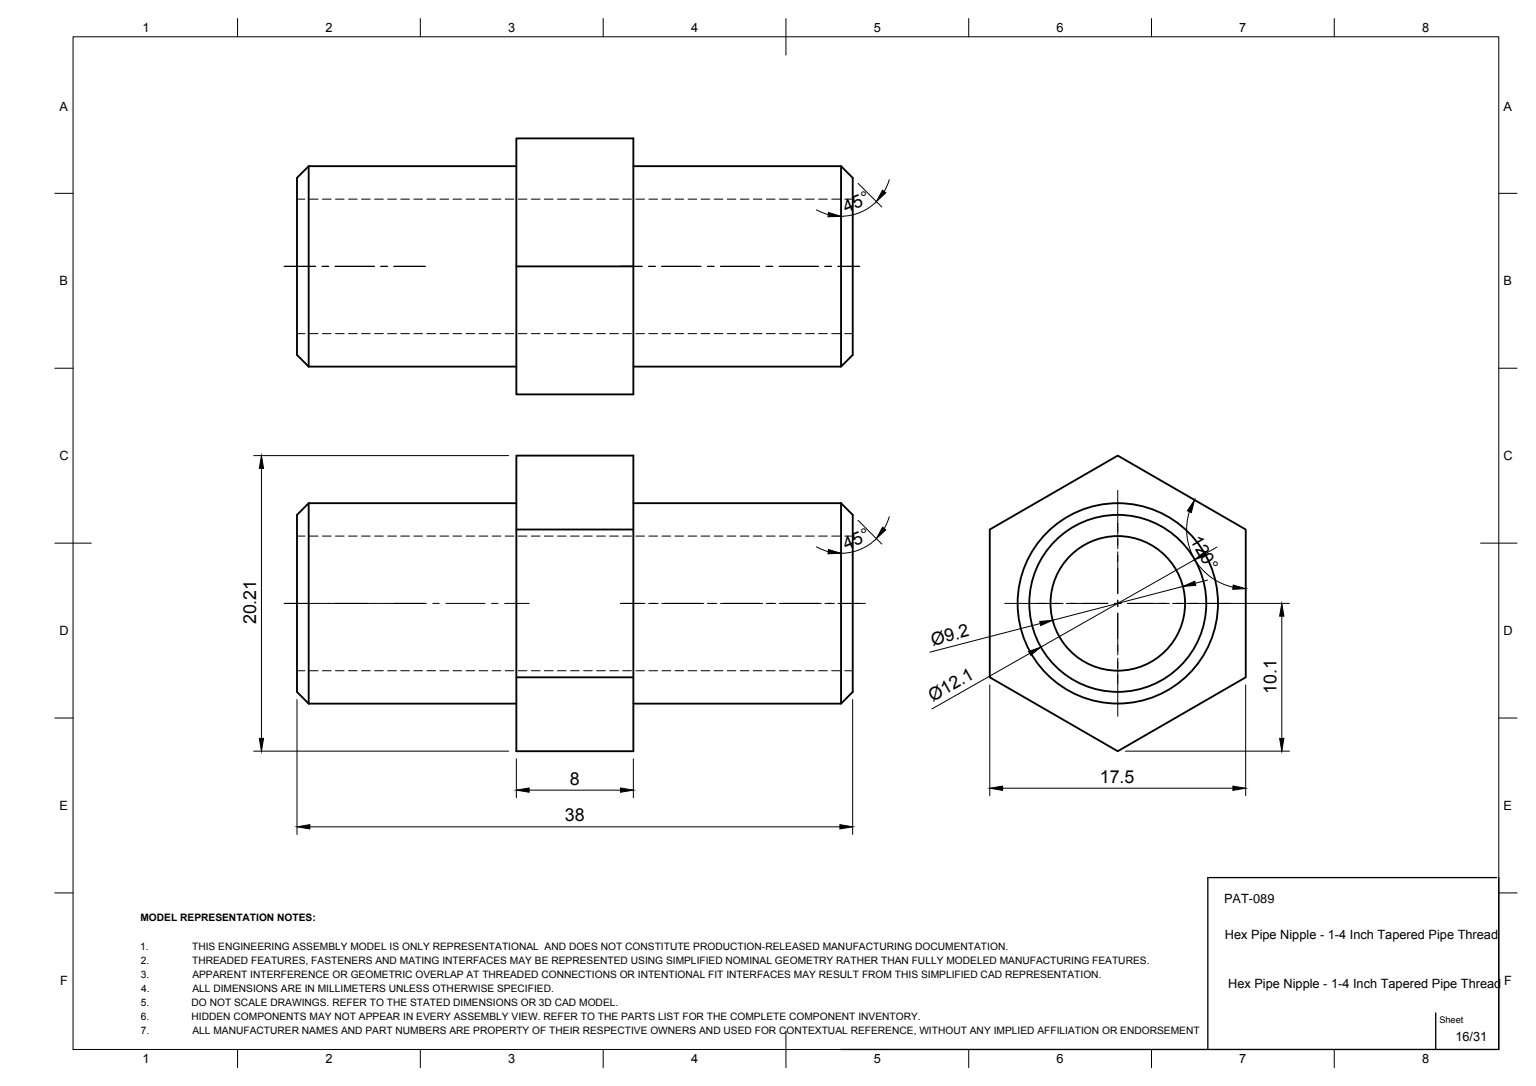
ISO-10303-21;
HEADER;
/* Generated by software containing ST-Developer
 * from STEP Tools, Inc. (www.steptools.com) 
 */

FILE_DESCRIPTION(
/* description */ ('Rotary union on bearing shaft'),
/* implementation_level */ '2;1');

FILE_NAME(
/* name */ 'Hex Pipe Nipple - 1-4 Inch Tapered Pipe Thread.step',
/* time_stamp */ '2026-10-28T03:24:01-07:00',
/* author */ (''),
/* organization */ (''),
/* preprocessor_version */ 'ST-DEVELOPER v20.2',
/* originating_system */ 'Autodesk Translation Framework v15.17.0.0',
/* authorisation */ '');

FILE_SCHEMA (('AUTOMOTIVE_DESIGN { 1 0 10303 214 3 1 1 }'));
ENDSEC;

DATA;
#10=MECHANICAL_DESIGN_GEOMETRIC_PRESENTATION_REPRESENTATION('',(#344),#9448);
#213=CONICAL_SURFACE('',#5729,0.645,0.785398163397448);
#214=CONICAL_SURFACE('',#5732,0.645,0.785398163397448);
#282=SHAPE_REPRESENTATION_RELATIONSHIP('SRR','None',#9584,#309);
#309=ADVANCED_BREP_SHAPE_REPRESENTATION('',(#377),#9444);
#344=STYLED_ITEM('',(#9771),#377);
#377=MANIFOLD_SOLID_BREP('Body1',#4901);
#481=FACE_BOUND('',#1302,.T.);
#482=FACE_BOUND('',#1304,.T.);
#483=FACE_BOUND('',#1313,.T.);
#484=FACE_BOUND('',#1318,.T.);
#616=PLANE('',#5714);
#617=PLANE('',#5716);
#618=PLANE('',#5718);
#619=PLANE('',#5719);
#620=PLANE('',#5720);
#621=PLANE('',#5721);
#622=PLANE('',#5722);
#623=PLANE('',#5723);
#624=PLANE('',#5726);
#625=PLANE('',#5734);
#901=FACE_OUTER_BOUND('',#1301,.T.);
#902=FACE_OUTER_BOUND('',#1303,.T.);
#903=FACE_OUTER_BOUND('',#1305,.T.);
#904=FACE_OUTER_BOUND('',#1306,.T.);
#905=FACE_OUTER_BOUND('',#1307,.T.);
#906=FACE_OUTER_BOUND('',#1308,.T.);
#907=FACE_OUTER_BOUND('',#1309,.T.);
#908=FACE_OUTER_BOUND('',#1310,.T.);
#909=FACE_OUTER_BOUND('',#1311,.T.);
#910=FACE_OUTER_BOUND('',#1312,.T.);
#911=FACE_OUTER_BOUND('',#1314,.T.);
#912=FACE_OUTER_BOUND('',#1315,.T.);
#913=FACE_OUTER_BOUND('',#1316,.T.);
#914=FACE_OUTER_BOUND('',#1317,.T.);
#915=FACE_OUTER_BOUND('',#1319,.T.);
#1301=EDGE_LOOP('',(#4255,#4256,#4257,#4258,#4259,#4260));
#1302=EDGE_LOOP('',(#4261));
#1303=EDGE_LOOP('',(#4262,#4263,#4264,#4265,#4266,#4267));
#1304=EDGE_LOOP('',(#4268));
#1305=EDGE_LOOP('',(#4269,#4270,#4271,#4272));
#1306=EDGE_LOOP('',(#4273,#4274,#4275,#4276));
#1307=EDGE_LOOP('',(#4277,#4278,#4279,#4280));
#1308=EDGE_LOOP('',(#4281,#4282,#4283,#4284));
#1309=EDGE_LOOP('',(#4285,#4286,#4287,#4288));
#1310=EDGE_LOOP('',(#4289,#4290,#4291,#4292));
#1311=EDGE_LOOP('',(#4293,#4294,#4295,#4296));
#1312=EDGE_LOOP('',(#4297));
#1313=EDGE_LOOP('',(#4298));
#1314=EDGE_LOOP('',(#4299,#4300,#4301,#4302));
#1315=EDGE_LOOP('',(#4303,#4304,#4305,#4306));
#1316=EDGE_LOOP('',(#4307,#4308,#4309,#4310));
#1317=EDGE_LOOP('',(#4311));
#1318=EDGE_LOOP('',(#4312));
#1319=EDGE_LOOP('',(#4313,#4314,#4315,#4316));
#1589=LINE('',#9110,#1909);
#1590=LINE('',#9112,#1910);
#1591=LINE('',#9114,#1911);
#1592=LINE('',#9116,#1912);
#1593=LINE('',#9118,#1913);
#1594=LINE('',#9119,#1914);
#1595=LINE('',#9125,#1915);
#1596=LINE('',#9127,#1916);
#1597=LINE('',#9129,#1917);
#1598=LINE('',#9131,#1918);
#1599=LINE('',#9133,#1919);
#1600=LINE('',#9134,#1920);
#1601=LINE('',#9138,#1921);
#1602=LINE('',#9139,#1922);
#1603=LINE('',#9141,#1923);
#1604=LINE('',#9143,#1924);
#1605=LINE('',#9145,#1925);
#1606=LINE('',#9147,#1926);
#1607=LINE('',#9151,#1927);
#1608=LINE('',#9159,#1928);
#1609=LINE('',#9163,#1929);
#1610=LINE('',#9167,#1930);
#1611=LINE('',#9172,#1931);
#1909=VECTOR('',#7078,1.);
#1910=VECTOR('',#7079,1.);
#1911=VECTOR('',#7080,1.);
#1912=VECTOR('',#7081,1.);
#1913=VECTOR('',#7082,1.);
#1914=VECTOR('',#7083,1.);
#1915=VECTOR('',#7088,1.);
#1916=VECTOR('',#7089,1.);
#1917=VECTOR('',#7090,1.);
#1918=VECTOR('',#7091,1.);
#1919=VECTOR('',#7092,1.);
#1920=VECTOR('',#7093,1.);
#1921=VECTOR('',#7098,1.);
#1922=VECTOR('',#7099,1.);
#1923=VECTOR('',#7102,1.);
#1924=VECTOR('',#7105,1.);
#1925=VECTOR('',#7108,1.);
#1926=VECTOR('',#7111,1.);
#1927=VECTOR('',#7116,0.685);
#1928=VECTOR('',#7127,0.645);
#1929=VECTOR('',#7132,0.685);
#1930=VECTOR('',#7137,0.645);
#1931=VECTOR('',#7144,0.46);
#2233=CIRCLE('',#5715,0.685);
#2234=CIRCLE('',#5717,0.685);
#2235=CIRCLE('',#5725,0.685);
#2236=CIRCLE('',#5727,0.605);
#2237=CIRCLE('',#5728,0.46);
#2238=CIRCLE('',#5731,0.685);
#2239=CIRCLE('',#5733,0.605);
#2240=CIRCLE('',#5735,0.46);
#2589=VERTEX_POINT('',#9108);
#2590=VERTEX_POINT('',#9109);
#2591=VERTEX_POINT('',#9111);
#2592=VERTEX_POINT('',#9113);
#2593=VERTEX_POINT('',#9115);
#2594=VERTEX_POINT('',#9117);
#2595=VERTEX_POINT('',#9120);
#2596=VERTEX_POINT('',#9123);
#2597=VERTEX_POINT('',#9124);
#2598=VERTEX_POINT('',#9126);
#2599=VERTEX_POINT('',#9128);
#2600=VERTEX_POINT('',#9130);
#2601=VERTEX_POINT('',#9132);
#2602=VERTEX_POINT('',#9135);
#2603=VERTEX_POINT('',#9150);
#2604=VERTEX_POINT('',#9154);
#2605=VERTEX_POINT('',#9156);
#2606=VERTEX_POINT('',#9161);
#2607=VERTEX_POINT('',#9165);
#2608=VERTEX_POINT('',#9169);
#3155=EDGE_CURVE('',#2589,#2590,#1589,.T.);
#3156=EDGE_CURVE('',#2590,#2591,#1590,.T.);
#3157=EDGE_CURVE('',#2591,#2592,#1591,.T.);
#3158=EDGE_CURVE('',#2592,#2593,#1592,.T.);
#3159=EDGE_CURVE('',#2593,#2594,#1593,.T.);
#3160=EDGE_CURVE('',#2594,#2589,#1594,.T.);
#3161=EDGE_CURVE('',#2595,#2595,#2233,.T.);
#3162=EDGE_CURVE('',#2596,#2597,#1595,.T.);
#3163=EDGE_CURVE('',#2597,#2598,#1596,.T.);
#3164=EDGE_CURVE('',#2598,#2599,#1597,.T.);
#3165=EDGE_CURVE('',#2599,#2600,#1598,.T.);
#3166=EDGE_CURVE('',#2600,#2601,#1599,.T.);
#3167=EDGE_CURVE('',#2601,#2596,#1600,.T.);
#3168=EDGE_CURVE('',#2602,#2602,#2234,.T.);
#3169=EDGE_CURVE('',#2596,#2590,#1601,.T.);
#3170=EDGE_CURVE('',#2591,#2601,#1602,.T.);
#3171=EDGE_CURVE('',#2592,#2600,#1603,.T.);
#3172=EDGE_CURVE('',#2593,#2599,#1604,.T.);
#3173=EDGE_CURVE('',#2594,#2598,#1605,.T.);
#3174=EDGE_CURVE('',#2589,#2597,#1606,.T.);
#3175=EDGE_CURVE('',#2602,#2603,#1607,.T.);
#3176=EDGE_CURVE('',#2603,#2603,#2235,.T.);
#3177=EDGE_CURVE('',#2604,#2604,#2236,.T.);
#3178=EDGE_CURVE('',#2605,#2605,#2237,.T.);
#3179=EDGE_CURVE('',#2603,#2604,#1608,.T.);
#3180=EDGE_CURVE('',#2606,#2606,#2238,.T.);
#3181=EDGE_CURVE('',#2606,#2595,#1609,.T.);
#3182=EDGE_CURVE('',#2607,#2607,#2239,.T.);
#3183=EDGE_CURVE('',#2607,#2606,#1610,.T.);
#3184=EDGE_CURVE('',#2608,#2608,#2240,.T.);
#3185=EDGE_CURVE('',#2608,#2605,#1611,.T.);
#4255=ORIENTED_EDGE('',*,*,#3155,.T.);
#4256=ORIENTED_EDGE('',*,*,#3156,.T.);
#4257=ORIENTED_EDGE('',*,*,#3157,.T.);
#4258=ORIENTED_EDGE('',*,*,#3158,.T.);
#4259=ORIENTED_EDGE('',*,*,#3159,.T.);
#4260=ORIENTED_EDGE('',*,*,#3160,.T.);
#4261=ORIENTED_EDGE('',*,*,#3161,.F.);
#4262=ORIENTED_EDGE('',*,*,#3162,.T.);
#4263=ORIENTED_EDGE('',*,*,#3163,.T.);
#4264=ORIENTED_EDGE('',*,*,#3164,.T.);
#4265=ORIENTED_EDGE('',*,*,#3165,.T.);
#4266=ORIENTED_EDGE('',*,*,#3166,.T.);
#4267=ORIENTED_EDGE('',*,*,#3167,.T.);
#4268=ORIENTED_EDGE('',*,*,#3168,.F.);
#4269=ORIENTED_EDGE('',*,*,#3169,.F.);
#4270=ORIENTED_EDGE('',*,*,#3167,.F.);
#4271=ORIENTED_EDGE('',*,*,#3170,.F.);
#4272=ORIENTED_EDGE('',*,*,#3156,.F.);
#4273=ORIENTED_EDGE('',*,*,#3170,.T.);
#4274=ORIENTED_EDGE('',*,*,#3166,.F.);
#4275=ORIENTED_EDGE('',*,*,#3171,.F.);
#4276=ORIENTED_EDGE('',*,*,#3157,.F.);
#4277=ORIENTED_EDGE('',*,*,#3171,.T.);
#4278=ORIENTED_EDGE('',*,*,#3165,.F.);
#4279=ORIENTED_EDGE('',*,*,#3172,.F.);
#4280=ORIENTED_EDGE('',*,*,#3158,.F.);
#4281=ORIENTED_EDGE('',*,*,#3172,.T.);
#4282=ORIENTED_EDGE('',*,*,#3164,.F.);
#4283=ORIENTED_EDGE('',*,*,#3173,.F.);
#4284=ORIENTED_EDGE('',*,*,#3159,.F.);
#4285=ORIENTED_EDGE('',*,*,#3173,.T.);
#4286=ORIENTED_EDGE('',*,*,#3163,.F.);
#4287=ORIENTED_EDGE('',*,*,#3174,.F.);
#4288=ORIENTED_EDGE('',*,*,#3160,.F.);
#4289=ORIENTED_EDGE('',*,*,#3174,.T.);
#4290=ORIENTED_EDGE('',*,*,#3162,.F.);
#4291=ORIENTED_EDGE('',*,*,#3169,.T.);
#4292=ORIENTED_EDGE('',*,*,#3155,.F.);
#4293=ORIENTED_EDGE('',*,*,#3168,.T.);
#4294=ORIENTED_EDGE('',*,*,#3175,.T.);
#4295=ORIENTED_EDGE('',*,*,#3176,.T.);
#4296=ORIENTED_EDGE('',*,*,#3175,.F.);
#4297=ORIENTED_EDGE('',*,*,#3177,.F.);
#4298=ORIENTED_EDGE('',*,*,#3178,.T.);
#4299=ORIENTED_EDGE('',*,*,#3176,.F.);
#4300=ORIENTED_EDGE('',*,*,#3179,.T.);
#4301=ORIENTED_EDGE('',*,*,#3177,.T.);
#4302=ORIENTED_EDGE('',*,*,#3179,.F.);
#4303=ORIENTED_EDGE('',*,*,#3180,.F.);
#4304=ORIENTED_EDGE('',*,*,#3181,.T.);
#4305=ORIENTED_EDGE('',*,*,#3161,.T.);
#4306=ORIENTED_EDGE('',*,*,#3181,.F.);
#4307=ORIENTED_EDGE('',*,*,#3182,.F.);
#4308=ORIENTED_EDGE('',*,*,#3183,.T.);
#4309=ORIENTED_EDGE('',*,*,#3180,.T.);
#4310=ORIENTED_EDGE('',*,*,#3183,.F.);
#4311=ORIENTED_EDGE('',*,*,#3182,.T.);
#4312=ORIENTED_EDGE('',*,*,#3184,.F.);
#4313=ORIENTED_EDGE('',*,*,#3184,.T.);
#4314=ORIENTED_EDGE('',*,*,#3185,.T.);
#4315=ORIENTED_EDGE('',*,*,#3178,.F.);
#4316=ORIENTED_EDGE('',*,*,#3185,.F.);
#4563=CYLINDRICAL_SURFACE('',#5724,0.685);
#4564=CYLINDRICAL_SURFACE('',#5730,0.685);
#4565=CYLINDRICAL_SURFACE('',#5736,0.46);
#4814=ADVANCED_FACE('',(#901,#481),#616,.F.);
#4815=ADVANCED_FACE('',(#902,#482),#617,.T.);
#4816=ADVANCED_FACE('',(#903),#618,.T.);
#4817=ADVANCED_FACE('',(#904),#619,.T.);
#4818=ADVANCED_FACE('',(#905),#620,.T.);
#4819=ADVANCED_FACE('',(#906),#621,.T.);
#4820=ADVANCED_FACE('',(#907),#622,.T.);
#4821=ADVANCED_FACE('',(#908),#623,.T.);
#4822=ADVANCED_FACE('',(#909),#4563,.T.);
#4823=ADVANCED_FACE('',(#910,#483),#624,.T.);
#4824=ADVANCED_FACE('',(#911),#213,.T.);
#4825=ADVANCED_FACE('',(#912),#4564,.T.);
#4826=ADVANCED_FACE('',(#913),#214,.T.);
#4827=ADVANCED_FACE('',(#914,#484),#625,.T.);
#4828=ADVANCED_FACE('',(#915),#4565,.F.);
#4901=CLOSED_SHELL('',(#4814,#4815,#4816,#4817,#4818,#4819,#4820,#4821,
#4822,#4823,#4824,#4825,#4826,#4827,#4828));
#5713=AXIS2_PLACEMENT_3D('',#9106,#7074,#7075);
#5714=AXIS2_PLACEMENT_3D('',#9107,#7076,#7077);
#5715=AXIS2_PLACEMENT_3D('',#9121,#7084,#7085);
#5716=AXIS2_PLACEMENT_3D('',#9122,#7086,#7087);
#5717=AXIS2_PLACEMENT_3D('',#9136,#7094,#7095);
#5718=AXIS2_PLACEMENT_3D('',#9137,#7096,#7097);
#5719=AXIS2_PLACEMENT_3D('',#9140,#7100,#7101);
#5720=AXIS2_PLACEMENT_3D('',#9142,#7103,#7104);
#5721=AXIS2_PLACEMENT_3D('',#9144,#7106,#7107);
#5722=AXIS2_PLACEMENT_3D('',#9146,#7109,#7110);
#5723=AXIS2_PLACEMENT_3D('',#9148,#7112,#7113);
#5724=AXIS2_PLACEMENT_3D('',#9149,#7114,#7115);
#5725=AXIS2_PLACEMENT_3D('',#9152,#7117,#7118);
#5726=AXIS2_PLACEMENT_3D('',#9153,#7119,#7120);
#5727=AXIS2_PLACEMENT_3D('',#9155,#7121,#7122);
#5728=AXIS2_PLACEMENT_3D('',#9157,#7123,#7124);
#5729=AXIS2_PLACEMENT_3D('',#9158,#7125,#7126);
#5730=AXIS2_PLACEMENT_3D('',#9160,#7128,#7129);
#5731=AXIS2_PLACEMENT_3D('',#9162,#7130,#7131);
#5732=AXIS2_PLACEMENT_3D('',#9164,#7133,#7134);
#5733=AXIS2_PLACEMENT_3D('',#9166,#7135,#7136);
#5734=AXIS2_PLACEMENT_3D('',#9168,#7138,#7139);
#5735=AXIS2_PLACEMENT_3D('',#9170,#7140,#7141);
#5736=AXIS2_PLACEMENT_3D('',#9171,#7142,#7143);
#7074=DIRECTION('axis',(0.,0.,1.));
#7075=DIRECTION('refdir',(1.,0.,0.));
#7076=DIRECTION('center_axis',(0.,1.,0.));
#7077=DIRECTION('ref_axis',(1.,0.,0.));
#7078=DIRECTION('',(-0.5,0.,0.866025403784439));
#7079=DIRECTION('',(-1.,0.,-3.29650746237182E-16));
#7080=DIRECTION('',(-0.5,0.,-0.866025403784439));
#7081=DIRECTION('',(0.5,0.,-0.866025403784438));
#7082=DIRECTION('',(1.,0.,0.));
#7083=DIRECTION('',(0.5,0.,0.866025403784439));
#7084=DIRECTION('center_axis',(0.,-1.,0.));
#7085=DIRECTION('ref_axis',(1.,0.,0.));
#7086=DIRECTION('center_axis',(0.,1.,0.));
#7087=DIRECTION('ref_axis',(1.,0.,0.));
#7088=DIRECTION('',(0.5,0.,-0.866025403784439));
#7089=DIRECTION('',(-0.5,0.,-0.866025403784439));
#7090=DIRECTION('',(-1.,0.,0.));
#7091=DIRECTION('',(-0.5,0.,0.866025403784438));
#7092=DIRECTION('',(0.5,0.,0.866025403784439));
#7093=DIRECTION('',(1.,0.,3.29650746237182E-16));
#7094=DIRECTION('center_axis',(0.,1.,0.));
#7095=DIRECTION('ref_axis',(1.,0.,0.));
#7096=DIRECTION('center_axis',(-3.29650746237182E-16,0.,1.));
#7097=DIRECTION('ref_axis',(1.,0.,3.29650746237182E-16));
#7098=DIRECTION('',(0.,-1.,0.));
#7099=DIRECTION('',(0.,1.,0.));
#7100=DIRECTION('center_axis',(-0.866025403784439,0.,0.5));
#7101=DIRECTION('ref_axis',(0.5,0.,0.866025403784439));
#7102=DIRECTION('',(0.,1.,0.));
#7103=DIRECTION('center_axis',(-0.866025403784439,0.,-0.5));
#7104=DIRECTION('ref_axis',(-0.5,0.,0.866025403784439));
#7105=DIRECTION('',(0.,1.,0.));
#7106=DIRECTION('center_axis',(0.,0.,-1.));
#7107=DIRECTION('ref_axis',(-1.,0.,0.));
#7108=DIRECTION('',(0.,1.,0.));
#7109=DIRECTION('center_axis',(0.866025403784439,0.,-0.5));
#7110=DIRECTION('ref_axis',(-0.5,0.,-0.866025403784439));
#7111=DIRECTION('',(0.,1.,0.));
#7112=DIRECTION('center_axis',(0.866025403784439,0.,0.5));
#7113=DIRECTION('ref_axis',(0.5,0.,-0.866025403784439));
#7114=DIRECTION('center_axis',(0.,-1.,0.));
#7115=DIRECTION('ref_axis',(1.,0.,0.));
#7116=DIRECTION('',(0.,1.,0.));
#7117=DIRECTION('center_axis',(0.,-1.,0.));
#7118=DIRECTION('ref_axis',(1.,0.,0.));
#7119=DIRECTION('center_axis',(0.,1.,0.));
#7120=DIRECTION('ref_axis',(0.,0.,1.));
#7121=DIRECTION('center_axis',(0.,-1.,0.));
#7122=DIRECTION('ref_axis',(1.,0.,0.));
#7123=DIRECTION('center_axis',(0.,-1.,0.));
#7124=DIRECTION('ref_axis',(1.,0.,0.));
#7125=DIRECTION('center_axis',(0.,-1.,0.));
#7126=DIRECTION('ref_axis',(1.,0.,0.));
#7127=DIRECTION('',(0.707106781186547,0.707106781186548,8.65956056235493E-17));
#7128=DIRECTION('center_axis',(0.,-1.,0.));
#7129=DIRECTION('ref_axis',(1.,0.,0.));
#7130=DIRECTION('center_axis',(0.,-1.,0.));
#7131=DIRECTION('ref_axis',(1.,0.,0.));
#7132=DIRECTION('',(0.,1.,0.));
#7133=DIRECTION('center_axis',(0.,1.,0.));
#7134=DIRECTION('ref_axis',(1.,0.,0.));
#7135=DIRECTION('center_axis',(0.,-1.,0.));
#7136=DIRECTION('ref_axis',(1.,0.,0.));
#7137=DIRECTION('',(-0.707106781186547,0.707106781186548,-8.65956056235493E-17));
#7138=DIRECTION('center_axis',(0.,-1.,0.));
#7139=DIRECTION('ref_axis',(0.,0.,-1.));
#7140=DIRECTION('center_axis',(0.,-1.,0.));
#7141=DIRECTION('ref_axis',(1.,0.,0.));
#7142=DIRECTION('center_axis',(0.,-1.,0.));
#7143=DIRECTION('ref_axis',(1.,0.,0.));
#7144=DIRECTION('',(0.,1.,0.));
#9106=CARTESIAN_POINT('',(0.,0.,0.));
#9107=CARTESIAN_POINT('Origin',(0.,-0.4,0.));
#9108=CARTESIAN_POINT('',(1.01036297108185,-0.4,0.));
#9109=CARTESIAN_POINT('',(0.505181485540923,-0.4,0.875));
#9110=CARTESIAN_POINT('',(0.505181485540923,-0.4,0.875));
#9111=CARTESIAN_POINT('',(-0.505181485540923,-0.4,0.875));
#9112=CARTESIAN_POINT('',(-0.505181485540923,-0.4,0.875));
#9113=CARTESIAN_POINT('',(-1.01036297108185,-0.4,-1.23733777851239E-16));
#9114=CARTESIAN_POINT('',(-1.01036297108185,-0.4,-1.23733777851239E-16));
#9115=CARTESIAN_POINT('',(-0.505181485540922,-0.4,-0.875));
#9116=CARTESIAN_POINT('',(-0.505181485540922,-0.4,-0.875));
#9117=CARTESIAN_POINT('',(0.505181485540923,-0.4,-0.875));
#9118=CARTESIAN_POINT('',(0.505181485540923,-0.4,-0.875));
#9119=CARTESIAN_POINT('',(1.01036297108185,-0.4,0.));
#9120=CARTESIAN_POINT('',(-0.685,-0.4,-8.38883057415937E-17));
#9121=CARTESIAN_POINT('Origin',(0.,-0.4,0.));
#9122=CARTESIAN_POINT('Origin',(0.,0.4,0.));
#9123=CARTESIAN_POINT('',(0.505181485540923,0.4,0.875));
#9124=CARTESIAN_POINT('',(1.01036297108185,0.4,0.));
#9125=CARTESIAN_POINT('',(0.505181485540923,0.4,0.875));
#9126=CARTESIAN_POINT('',(0.505181485540923,0.4,-0.875));
#9127=CARTESIAN_POINT('',(1.01036297108185,0.4,0.));
#9128=CARTESIAN_POINT('',(-0.505181485540922,0.4,-0.875));
#9129=CARTESIAN_POINT('',(0.505181485540923,0.4,-0.875));
#9130=CARTESIAN_POINT('',(-1.01036297108185,0.4,-1.23733777851239E-16));
#9131=CARTESIAN_POINT('',(-0.505181485540922,0.4,-0.875));
#9132=CARTESIAN_POINT('',(-0.505181485540923,0.4,0.875));
#9133=CARTESIAN_POINT('',(-1.01036297108185,0.4,-1.23733777851239E-16));
#9134=CARTESIAN_POINT('',(-0.505181485540923,0.4,0.875));
#9135=CARTESIAN_POINT('',(-0.685,0.4,8.38883057415937E-17));
#9136=CARTESIAN_POINT('Origin',(0.,0.4,0.));
#9137=CARTESIAN_POINT('Origin',(-0.505181485540923,0.,0.875));
#9138=CARTESIAN_POINT('',(0.505181485540923,0.,0.875));
#9139=CARTESIAN_POINT('',(-0.505181485540923,0.,0.875));
#9140=CARTESIAN_POINT('Origin',(-1.01036297108185,0.,-1.23733777851239E-16));
#9141=CARTESIAN_POINT('',(-1.01036297108185,0.,-1.23733777851239E-16));
#9142=CARTESIAN_POINT('Origin',(-0.505181485540922,0.,-0.875));
#9143=CARTESIAN_POINT('',(-0.505181485540922,0.,-0.875));
#9144=CARTESIAN_POINT('Origin',(0.505181485540923,0.,-0.875));
#9145=CARTESIAN_POINT('',(0.505181485540923,0.,-0.875));
#9146=CARTESIAN_POINT('Origin',(1.01036297108185,0.,0.));
#9147=CARTESIAN_POINT('',(1.01036297108185,0.,0.));
#9148=CARTESIAN_POINT('Origin',(0.505181485540923,0.,0.875));
#9149=CARTESIAN_POINT('Origin',(0.,0.,0.));
#9150=CARTESIAN_POINT('',(-0.685,1.82,-8.38883057415937E-17));
#9151=CARTESIAN_POINT('',(-0.685,0.,-8.38883057415937E-17));
#9152=CARTESIAN_POINT('Origin',(0.,1.82,0.));
#9153=CARTESIAN_POINT('Origin',(0.605,1.9,0.));
#9154=CARTESIAN_POINT('',(-0.605,1.9,-7.40911313484149E-17));
#9155=CARTESIAN_POINT('Origin',(0.,1.9,0.));
#9156=CARTESIAN_POINT('',(-0.46,1.9,-5.63337527607782E-17));
#9157=CARTESIAN_POINT('Origin',(0.,1.9,0.));
#9158=CARTESIAN_POINT('Origin',(0.,1.86,0.));
#9159=CARTESIAN_POINT('',(-0.645,1.86,-7.89897185450043E-17));
#9160=CARTESIAN_POINT('Origin',(0.,0.,0.));
#9161=CARTESIAN_POINT('',(-0.685,-1.82,-8.38883057415937E-17));
#9162=CARTESIAN_POINT('Origin',(0.,-1.82,0.));
#9163=CARTESIAN_POINT('',(-0.685,0.,-8.38883057415937E-17));
#9164=CARTESIAN_POINT('Origin',(0.,-1.86,0.));
#9165=CARTESIAN_POINT('',(-0.605,-1.9,-7.40911313484149E-17));
#9166=CARTESIAN_POINT('Origin',(0.,-1.9,0.));
#9167=CARTESIAN_POINT('',(-0.645,-1.86,-7.89897185450043E-17));
#9168=CARTESIAN_POINT('Origin',(0.46,-1.9,0.));
#9169=CARTESIAN_POINT('',(-0.46,-1.9,-5.63337527607782E-17));
#9170=CARTESIAN_POINT('Origin',(0.,-1.9,0.));
#9171=CARTESIAN_POINT('Origin',(0.,0.,0.));
#9172=CARTESIAN_POINT('',(-0.46,0.,-5.63337527607782E-17));
#9412=UNCERTAINTY_MEASURE_WITH_UNIT(LENGTH_MEASURE(0.001),#9449,
'DISTANCE_ACCURACY_VALUE',
'Maximum model space distance between geometric entities at asserted c
onnectivities');
#9416=UNCERTAINTY_MEASURE_WITH_UNIT(LENGTH_MEASURE(0.001),#9449,
'DISTANCE_ACCURACY_VALUE',
'Maximum model space distance between geometric entities at asserted c
onnectivities');
#9444=(
GEOMETRIC_REPRESENTATION_CONTEXT(3)
GLOBAL_UNCERTAINTY_ASSIGNED_CONTEXT((#9412))
GLOBAL_UNIT_ASSIGNED_CONTEXT((#9449,#9451,#9452))
REPRESENTATION_CONTEXT('','3D')
);
#9448=(
GEOMETRIC_REPRESENTATION_CONTEXT(3)
GLOBAL_UNCERTAINTY_ASSIGNED_CONTEXT((#9416))
GLOBAL_UNIT_ASSIGNED_CONTEXT((#9449,#9451,#9452))
REPRESENTATION_CONTEXT('','3D')
);
#9449=(
LENGTH_UNIT()
NAMED_UNIT(*)
SI_UNIT(.CENTI.,.METRE.)
);
#9451=(
NAMED_UNIT(*)
PLANE_ANGLE_UNIT()
SI_UNIT($,.RADIAN.)
);
#9452=(
NAMED_UNIT(*)
SI_UNIT($,.STERADIAN.)
SOLID_ANGLE_UNIT()
);
#9480=SHAPE_DEFINITION_REPRESENTATION(#9516,#9584);
#9516=PRODUCT_DEFINITION_SHAPE('',$,#9616);
#9584=SHAPE_REPRESENTATION('',(#5713),#9444);
#9588=PRODUCT_DEFINITION_CONTEXT('part definition',#9683,'design');
#9616=PRODUCT_DEFINITION(
'Hex Pipe Nipple - 1-4 Inch Tapered Pipe Thread',
'Hex Pipe Nipple - 1-4 Inch Tapered Pipe Thread',#9647,#9588);
#9647=PRODUCT_DEFINITION_FORMATION('',$,#9712);
#9683=APPLICATION_CONTEXT(
'Core Data for Automotive Mechanical Design Process');
#9684=PRODUCT_CONTEXT('part definition',#9683,'mechanical');
#9712=PRODUCT('Hex Pipe Nipple - 1-4 Inch Tapered Pipe Thread',
'Hex Pipe Nipple - 1-4 Inch Tapered Pipe Thread',
'Hex Pipe Nipple - 1-4 Inch Tapered Pipe Thread',(#9684));
#9765=COLOUR_RGB('Sky Blue',0.24,0.69,0.87);
#9766=FILL_AREA_STYLE_COLOUR('',#9765);
#9767=FILL_AREA_STYLE('',(#9766));
#9768=SURFACE_STYLE_FILL_AREA(#9767);
#9769=SURFACE_SIDE_STYLE('',(#9768));
#9770=SURFACE_STYLE_USAGE(.BOTH.,#9769);
#9771=PRESENTATION_STYLE_ASSIGNMENT((#9770));
ENDSEC;
END-ISO-10303-21;
